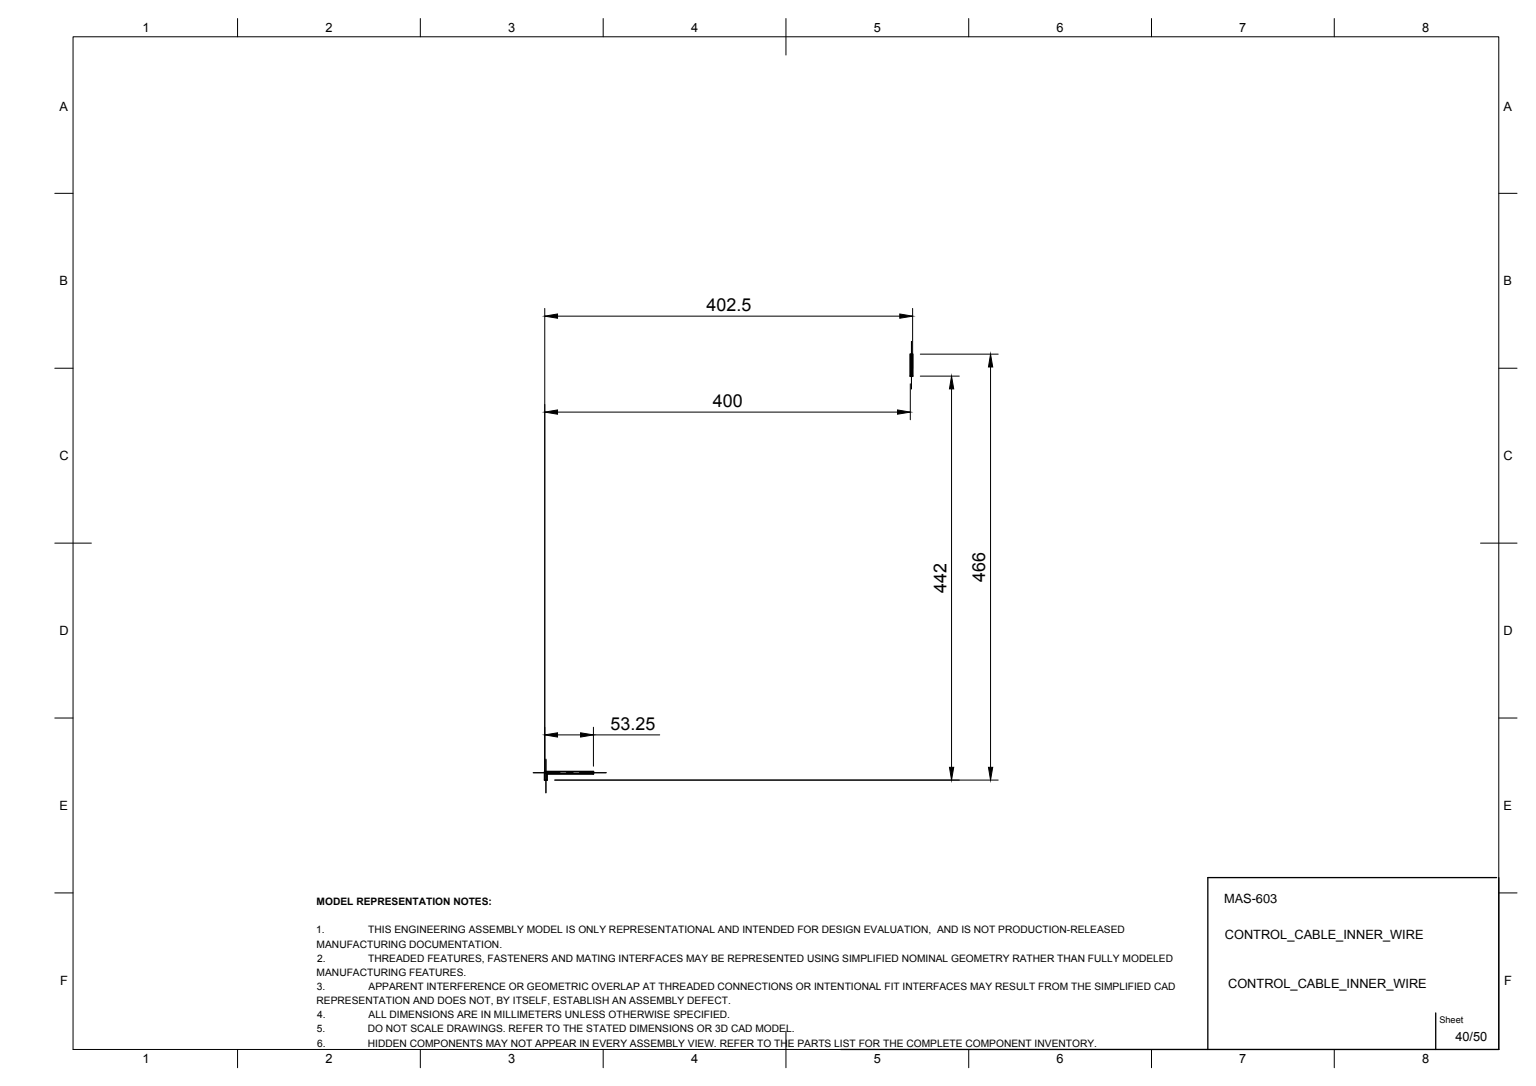
ISO-10303-21;
HEADER;
FILE_DESCRIPTION((''),'2;1');
FILE_NAME('CONTROL_CABLE_INNER_WIRE.step','2026-10-01T22:06:14-07:00',(''),(''),'','','');
FILE_SCHEMA (('AUTOMOTIVE_DESIGN { 1 0 10303 214 3 1 1 }'));
ENDSEC;
DATA;
#10=MECHANICAL_DESIGN_GEOMETRIC_PRESENTATION_REPRESENTATION('',(#1013,#1014),#50440);
#413=ELLIPSE('',#31038,0.176776695296637,0.125) ;
#414=ELLIPSE('',#31039,0.176776695296637,0.125) ;
#415=ELLIPSE('',#31041,0.176776695296637,0.125) ;
#416=ELLIPSE('',#31042,0.176776695296637,0.125) ;
#920=SHAPE_REPRESENTATION_RELATIONSHIP('SRR','None',#50653,#965) ;
#965=ADVANCED_BREP_SHAPE_REPRESENTATION('',(#1067,#1068),#50422) ;
#1013=STYLED_ITEM('',(#50883),#1067) ;
#1014=STYLED_ITEM('',(#50883),#1068) ;
#1067=MANIFOLD_SOLID_BREP('CONTROL_CABLE_INNER_WIRE',#28689) ;
#1068=MANIFOLD_SOLID_BREP('CONTROL_CABLE_INNER_WIRE',#28690) ;
#2234=PLANE('',#31044) ;
#2235=PLANE('',#31045) ;
#2236=PLANE('',#31046) ;
#2237=PLANE('',#31051) ;
#2238=PLANE('',#31055) ;
#2239=PLANE('',#31056) ;
#3460=FACE_OUTER_BOUND('',#5281,.T.) ;
#3461=FACE_OUTER_BOUND('',#5282,.T.) ;
#3462=FACE_OUTER_BOUND('',#5283,.T.) ;
#3463=FACE_OUTER_BOUND('',#5284,.T.) ;
#3464=FACE_OUTER_BOUND('',#5285,.T.) ;
#3465=FACE_OUTER_BOUND('',#5286,.T.) ;
#3466=FACE_OUTER_BOUND('',#5287,.T.) ;
#3467=FACE_OUTER_BOUND('',#5288,.T.) ;
#3468=FACE_OUTER_BOUND('',#5289,.T.) ;
#5281=EDGE_LOOP('',(#24249,#24250,#24251,#24252,#24253,#24254,#24255,#24256)) ;
#5282=EDGE_LOOP('',(#24257)) ;
#5283=EDGE_LOOP('',(#24258,#24259,#24260,#24261)) ;
#5284=EDGE_LOOP('',(#24262,#24263,#24264)) ;
#5285=EDGE_LOOP('',(#24265,#24266,#24267,#24268,#24269,#24270,#24271,#24272,
#24273,#24274,#24275)) ;
#5286=EDGE_LOOP('',(#24276)) ;
#5287=EDGE_LOOP('',(#24277,#24278,#24279,#24280)) ;
#5288=EDGE_LOOP('',(#24281)) ;
#5289=EDGE_LOOP('',(#24282)) ;
#7893=LINE('',#47471,#10365) ;
#7894=LINE('',#47481,#10366) ;
#7895=LINE('',#47483,#10367) ;
#7896=LINE('',#47484,#10368) ;
#7897=LINE('',#47491,#10369) ;
#7898=LINE('',#47498,#10370) ;
#10365=VECTOR('',#38198,0.125) ;
#10366=VECTOR('',#38211,1.) ;
#10367=VECTOR('',#38212,1.) ;
#10368=VECTOR('',#38213,1.) ;
#10369=VECTOR('',#38222,0.125) ;
#10370=VECTOR('',#38231,0.125) ;
#11284=CIRCLE('',#31040,0.125) ;
#11285=CIRCLE('',#31043,0.125) ;
#11286=CIRCLE('',#31047,0.125) ;
#11287=CIRCLE('',#31048,0.125) ;
#11288=CIRCLE('',#31050,0.125) ;
#11289=CIRCLE('',#31053,0.125) ;
#11290=CIRCLE('',#31054,0.125) ;
#13737=VERTEX_POINT('',#47465) ;
#13738=VERTEX_POINT('',#47466) ;
#13739=VERTEX_POINT('',#47468) ;
#13740=VERTEX_POINT('',#47470) ;
#13741=VERTEX_POINT('',#47473) ;
#13742=VERTEX_POINT('',#47475) ;
#13743=VERTEX_POINT('',#47480) ;
#13744=VERTEX_POINT('',#47482) ;
#13745=VERTEX_POINT('',#47486) ;
#13746=VERTEX_POINT('',#47490) ;
#13747=VERTEX_POINT('',#47495) ;
#13748=VERTEX_POINT('',#47497) ;
#17390=EDGE_CURVE('',#13737,#13738,#413,.T.) ;
#17391=EDGE_CURVE('',#13739,#13737,#414,.T.) ;
#17392=EDGE_CURVE('',#13739,#13740,#7893,.T.) ;
#17393=EDGE_CURVE('',#13740,#13740,#11284,.T.) ;
#17394=EDGE_CURVE('',#13741,#13739,#415,.T.) ;
#17395=EDGE_CURVE('',#13742,#13741,#416,.T.) ;
#17396=EDGE_CURVE('',#13738,#13742,#11285,.T.) ;
#17397=EDGE_CURVE('',#13738,#13743,#7894,.T.) ;
#17398=EDGE_CURVE('',#13744,#13742,#7895,.T.) ;
#17399=EDGE_CURVE('',#13743,#13744,#7896,.T.) ;
#17400=EDGE_CURVE('',#13744,#13745,#11286,.T.) ;
#17401=EDGE_CURVE('',#13745,#13743,#11287,.T.) ;
#17402=EDGE_CURVE('',#13745,#13746,#7897,.T.) ;
#17403=EDGE_CURVE('',#13746,#13746,#11288,.T.) ;
#17404=EDGE_CURVE('',#13747,#13747,#11289,.T.) ;
#17405=EDGE_CURVE('',#13747,#13748,#7898,.T.) ;
#17406=EDGE_CURVE('',#13748,#13748,#11290,.T.) ;
#24249=ORIENTED_EDGE('',*,*,#17390,.F.) ;
#24250=ORIENTED_EDGE('',*,*,#17391,.F.) ;
#24251=ORIENTED_EDGE('',*,*,#17392,.T.) ;
#24252=ORIENTED_EDGE('',*,*,#17393,.F.) ;
#24253=ORIENTED_EDGE('',*,*,#17392,.F.) ;
#24254=ORIENTED_EDGE('',*,*,#17394,.F.) ;
#24255=ORIENTED_EDGE('',*,*,#17395,.F.) ;
#24256=ORIENTED_EDGE('',*,*,#17396,.F.) ;
#24257=ORIENTED_EDGE('',*,*,#17393,.T.) ;
#24258=ORIENTED_EDGE('',*,*,#17397,.F.) ;
#24259=ORIENTED_EDGE('',*,*,#17396,.T.) ;
#24260=ORIENTED_EDGE('',*,*,#17398,.F.) ;
#24261=ORIENTED_EDGE('',*,*,#17399,.F.) ;
#24262=ORIENTED_EDGE('',*,*,#17399,.T.) ;
#24263=ORIENTED_EDGE('',*,*,#17400,.T.) ;
#24264=ORIENTED_EDGE('',*,*,#17401,.T.) ;
#24265=ORIENTED_EDGE('',*,*,#17397,.T.) ;
#24266=ORIENTED_EDGE('',*,*,#17401,.F.) ;
#24267=ORIENTED_EDGE('',*,*,#17402,.T.) ;
#24268=ORIENTED_EDGE('',*,*,#17403,.F.) ;
#24269=ORIENTED_EDGE('',*,*,#17402,.F.) ;
#24270=ORIENTED_EDGE('',*,*,#17400,.F.) ;
#24271=ORIENTED_EDGE('',*,*,#17398,.T.) ;
#24272=ORIENTED_EDGE('',*,*,#17395,.T.) ;
#24273=ORIENTED_EDGE('',*,*,#17394,.T.) ;
#24274=ORIENTED_EDGE('',*,*,#17391,.T.) ;
#24275=ORIENTED_EDGE('',*,*,#17390,.T.) ;
#24276=ORIENTED_EDGE('',*,*,#17403,.T.) ;
#24277=ORIENTED_EDGE('',*,*,#17404,.F.) ;
#24278=ORIENTED_EDGE('',*,*,#17405,.T.) ;
#24279=ORIENTED_EDGE('',*,*,#17406,.F.) ;
#24280=ORIENTED_EDGE('',*,*,#17405,.F.) ;
#24281=ORIENTED_EDGE('',*,*,#17406,.T.) ;
#24282=ORIENTED_EDGE('',*,*,#17404,.T.) ;
#26890=CYLINDRICAL_SURFACE('',#31037,0.125) ;
#26891=CYLINDRICAL_SURFACE('',#31049,0.125) ;
#26892=CYLINDRICAL_SURFACE('',#31052,0.125) ;
#28195=ADVANCED_FACE('',(#3460),#26890,.T.) ;
#28196=ADVANCED_FACE('',(#3461),#2234,.T.) ;
#28197=ADVANCED_FACE('',(#3462),#2235,.T.) ;
#28198=ADVANCED_FACE('',(#3463),#2236,.T.) ;
#28199=ADVANCED_FACE('',(#3464),#26891,.T.) ;
#28200=ADVANCED_FACE('',(#3465),#2237,.T.) ;
#28201=ADVANCED_FACE('',(#3466),#26892,.T.) ;
#28202=ADVANCED_FACE('',(#3467),#2238,.T.) ;
#28203=ADVANCED_FACE('',(#3468),#2239,.T.) ;
#28689=CLOSED_SHELL('',(#28195,#28196,#28197,#28198,#28199,#28200)) ;
#28690=CLOSED_SHELL('',(#28201,#28202,#28203)) ;
#31036=AXIS2_PLACEMENT_3D('',#47463,#38190,#38191) ;
#31037=AXIS2_PLACEMENT_3D('',#47464,#38192,#38193) ;
#31038=AXIS2_PLACEMENT_3D('',#47467,#38194,#38195) ;
#31039=AXIS2_PLACEMENT_3D('',#47469,#38196,#38197) ;
#31040=AXIS2_PLACEMENT_3D('',#47472,#38199,#38200) ;
#31041=AXIS2_PLACEMENT_3D('',#47474,#38201,#38202) ;
#31042=AXIS2_PLACEMENT_3D('',#47476,#38203,#38204) ;
#31043=AXIS2_PLACEMENT_3D('',#47477,#38205,#38206) ;
#31044=AXIS2_PLACEMENT_3D('',#47478,#38207,#38208) ;
#31045=AXIS2_PLACEMENT_3D('',#47479,#38209,#38210) ;
#31046=AXIS2_PLACEMENT_3D('',#47485,#38214,#38215) ;
#31047=AXIS2_PLACEMENT_3D('',#47487,#38216,#38217) ;
#31048=AXIS2_PLACEMENT_3D('',#47488,#38218,#38219) ;
#31049=AXIS2_PLACEMENT_3D('',#47489,#38220,#38221) ;
#31050=AXIS2_PLACEMENT_3D('',#47492,#38223,#38224) ;
#31051=AXIS2_PLACEMENT_3D('',#47493,#38225,#38226) ;
#31052=AXIS2_PLACEMENT_3D('',#47494,#38227,#38228) ;
#31053=AXIS2_PLACEMENT_3D('',#47496,#38229,#38230) ;
#31054=AXIS2_PLACEMENT_3D('',#47499,#38232,#38233) ;
#31055=AXIS2_PLACEMENT_3D('',#47500,#38234,#38235) ;
#31056=AXIS2_PLACEMENT_3D('',#47501,#38236,#38237) ;
#38190=DIRECTION('axis',(0.,0.,1.)) ;
#38191=DIRECTION('refdir',(1.,0.,0.)) ;
#38192=DIRECTION('center_axis',(0.,0.,1.)) ;
#38193=DIRECTION('ref_axis',(1.,0.,0.)) ;
#38194=DIRECTION('center_axis',(-0.707106781186548,0.,-0.707106781186548)) ;
#38195=DIRECTION('ref_axis',(0.707106781186547,0.,-0.707106781186547)) ;
#38196=DIRECTION('center_axis',(-0.707106781186548,0.,0.707106781186548)) ;
#38197=DIRECTION('ref_axis',(0.707106781186547,0.,0.707106781186547)) ;
#38198=DIRECTION('',(0.,0.,-1.)) ;
#38199=DIRECTION('center_axis',(0.,0.,-1.)) ;
#38200=DIRECTION('ref_axis',(1.,0.,0.)) ;
#38201=DIRECTION('center_axis',(-0.707106781186548,0.,0.707106781186548)) ;
#38202=DIRECTION('ref_axis',(0.707106781186547,0.,0.707106781186547)) ;
#38203=DIRECTION('center_axis',(-0.707106781186548,0.,-0.707106781186548)) ;
#38204=DIRECTION('ref_axis',(0.707106781186547,0.,-0.707106781186547)) ;
#38205=DIRECTION('center_axis',(0.,0.,1.)) ;
#38206=DIRECTION('ref_axis',(1.,0.,0.)) ;
#38207=DIRECTION('center_axis',(0.,0.,-1.)) ;
#38208=DIRECTION('ref_axis',(-1.,0.,0.)) ;
#38209=DIRECTION('center_axis',(0.,0.,1.)) ;
#38210=DIRECTION('ref_axis',(1.,0.,0.)) ;
#38211=DIRECTION('',(1.,0.,0.)) ;
#38212=DIRECTION('',(-1.,0.,0.)) ;
#38213=DIRECTION('',(0.,1.,0.)) ;
#38214=DIRECTION('center_axis',(1.,0.,0.)) ;
#38215=DIRECTION('ref_axis',(0.,0.,-1.)) ;
#38216=DIRECTION('center_axis',(1.,0.,0.)) ;
#38217=DIRECTION('ref_axis',(0.,0.,-1.)) ;
#38218=DIRECTION('center_axis',(1.,0.,0.)) ;
#38219=DIRECTION('ref_axis',(0.,0.,-1.)) ;
#38220=DIRECTION('center_axis',(1.,0.,0.)) ;
#38221=DIRECTION('ref_axis',(0.,0.,-1.)) ;
#38222=DIRECTION('',(-1.,0.,0.)) ;
#38223=DIRECTION('center_axis',(-1.,0.,0.)) ;
#38224=DIRECTION('ref_axis',(0.,0.,-1.)) ;
#38225=DIRECTION('center_axis',(-1.,0.,0.)) ;
#38226=DIRECTION('ref_axis',(0.,0.,1.)) ;
#38227=DIRECTION('center_axis',(0.,0.,1.)) ;
#38228=DIRECTION('ref_axis',(1.,0.,0.)) ;
#38229=DIRECTION('center_axis',(0.,0.,1.)) ;
#38230=DIRECTION('ref_axis',(1.,0.,0.)) ;
#38231=DIRECTION('',(0.,0.,-1.)) ;
#38232=DIRECTION('center_axis',(0.,0.,-1.)) ;
#38233=DIRECTION('ref_axis',(1.,0.,0.)) ;
#38234=DIRECTION('center_axis',(0.,0.,-1.)) ;
#38235=DIRECTION('ref_axis',(-1.,0.,0.)) ;
#38236=DIRECTION('center_axis',(0.,0.,1.)) ;
#38237=DIRECTION('ref_axis',(1.,0.,0.)) ;
#47463=CARTESIAN_POINT('',(0.,0.,0.)) ;
#47464=CARTESIAN_POINT('Origin',(-13.,0.,43.25)) ;
#47465=CARTESIAN_POINT('',(-13.,-0.125,43.6)) ;
#47466=CARTESIAN_POINT('',(-13.1,-0.0749999999999981,43.7)) ;
#47467=CARTESIAN_POINT('Origin',(-13.,0.,43.6)) ;
#47468=CARTESIAN_POINT('',(-13.125,-1.53080849893416E-17,43.475)) ;
#47469=CARTESIAN_POINT('Origin',(-13.,0.,43.6)) ;
#47470=CARTESIAN_POINT('',(-13.125,-1.53080849893419E-17,42.8)) ;
#47471=CARTESIAN_POINT('',(-13.125,-1.53080849893419E-17,43.25)) ;
#47472=CARTESIAN_POINT('Origin',(-13.,0.,42.8)) ;
#47473=CARTESIAN_POINT('',(-13.,0.125,43.6)) ;
#47474=CARTESIAN_POINT('Origin',(-13.,0.,43.6)) ;
#47475=CARTESIAN_POINT('',(-13.1,0.0749999999999981,43.7)) ;
#47476=CARTESIAN_POINT('Origin',(-13.,0.,43.6)) ;
#47477=CARTESIAN_POINT('Origin',(-13.,0.,43.7)) ;
#47478=CARTESIAN_POINT('Origin',(-13.,0.,42.8)) ;
#47479=CARTESIAN_POINT('Origin',(-13.,0.,43.7)) ;
#47480=CARTESIAN_POINT('',(-13.,-0.0749999999999981,43.7)) ;
#47481=CARTESIAN_POINT('',(-15.6,-0.0749999999999981,43.7)) ;
#47482=CARTESIAN_POINT('',(-13.,0.0749999999999981,43.7)) ;
#47483=CARTESIAN_POINT('',(-15.6,0.0749999999999981,43.7)) ;
#47484=CARTESIAN_POINT('',(-13.,0.,43.7)) ;
#47485=CARTESIAN_POINT('Origin',(-13.,0.,43.6)) ;
#47486=CARTESIAN_POINT('',(-13.,-1.53080849893419E-17,43.725)) ;
#47487=CARTESIAN_POINT('Origin',(-13.,0.,43.6)) ;
#47488=CARTESIAN_POINT('Origin',(-13.,0.,43.6)) ;
#47489=CARTESIAN_POINT('Origin',(-15.6,0.,43.6)) ;
#47490=CARTESIAN_POINT('',(-18.2,-1.53080849893419E-17,43.725)) ;
#47491=CARTESIAN_POINT('',(-15.6,-1.53080849893419E-17,43.725)) ;
#47492=CARTESIAN_POINT('Origin',(-18.2,0.,43.6)) ;
#47493=CARTESIAN_POINT('Origin',(-18.2,0.,43.6)) ;
#47494=CARTESIAN_POINT('Origin',(-53.,19.,88.2)) ;
#47495=CARTESIAN_POINT('',(-53.125,19.,89.4)) ;
#47496=CARTESIAN_POINT('Origin',(-53.,19.,89.4)) ;
#47497=CARTESIAN_POINT('',(-53.125,19.,87.)) ;
#47498=CARTESIAN_POINT('',(-53.125,19.,88.2)) ;
#47499=CARTESIAN_POINT('Origin',(-53.,19.,87.)) ;
#47500=CARTESIAN_POINT('Origin',(-53.,19.,87.)) ;
#47501=CARTESIAN_POINT('Origin',(-53.,19.,89.4)) ;
#50369=UNCERTAINTY_MEASURE_WITH_UNIT(LENGTH_MEASURE(0.001),#50441,
'DISTANCE_ACCURACY_VALUE',
'Maximum model space distance between geometric entities at asserted c
onnectivities') ;
#50387=UNCERTAINTY_MEASURE_WITH_UNIT(LENGTH_MEASURE(0.001),#50441,
'DISTANCE_ACCURACY_VALUE',
'Maximum model space distance between geometric entities at asserted c
onnectivities') ;
#50422=(
GEOMETRIC_REPRESENTATION_CONTEXT(3)
GLOBAL_UNCERTAINTY_ASSIGNED_CONTEXT((#50369))
GLOBAL_UNIT_ASSIGNED_CONTEXT((#50441,#50443,#50444))
REPRESENTATION_CONTEXT('','3D')
) ;
#50440=(
GEOMETRIC_REPRESENTATION_CONTEXT(3)
GLOBAL_UNCERTAINTY_ASSIGNED_CONTEXT((#50387))
GLOBAL_UNIT_ASSIGNED_CONTEXT((#50441,#50443,#50444))
REPRESENTATION_CONTEXT('','3D')
) ;
#50441=(
LENGTH_UNIT()
NAMED_UNIT(*)
SI_UNIT(.CENTI.,.METRE.)
) ;
#50443=(
NAMED_UNIT(*)
PLANE_ANGLE_UNIT()
SI_UNIT($,.RADIAN.)
) ;
#50444=(
NAMED_UNIT(*)
SI_UNIT($,.STERADIAN.)
SOLID_ANGLE_UNIT()
) ;
#50479=SHAPE_DEFINITION_REPRESENTATION(#50555,#50653) ;
#50555=PRODUCT_DEFINITION_SHAPE('',$,#50706) ;
#50653=SHAPE_REPRESENTATION('',(#31036),#50422) ;
#50671=PRODUCT_DEFINITION_CONTEXT('part definition',#50829,'design') ;
#50706=PRODUCT_DEFINITION('CONTROL_CABLE_INNER_WIRE',
'CONTROL_CABLE_INNER_WIRE',#50758,#50671) ;
#50758=PRODUCT_DEFINITION_FORMATION('',$,#50865) ;
#50829=APPLICATION_CONTEXT(
'Core Data for Automotive Mechanical Design Process') ;
#50830=PRODUCT_CONTEXT('part definition',#50829,'mechanical') ;
#50865=PRODUCT('CONTROL_CABLE_INNER_WIRE','CONTROL_CABLE_INNER_WIRE',$,(#50830)) ;
#50883=PRESENTATION_STYLE_ASSIGNMENT((#50890)) ;
#50890=SURFACE_STYLE_USAGE(.BOTH.,#50897) ;
#50897=SURFACE_SIDE_STYLE('',(#50904)) ;
#50904=SURFACE_STYLE_FILL_AREA(#50911) ;
#50911=FILL_AREA_STYLE('Steel - Satin',(#50918)) ;
#50918=FILL_AREA_STYLE_COLOUR('Steel - Satin',#50925) ;
#50925=COLOUR_RGB('Steel - Satin', 0.31764706, 0.68627451, 0.89019608) ;
ENDSEC;
END-ISO-10303-21;
